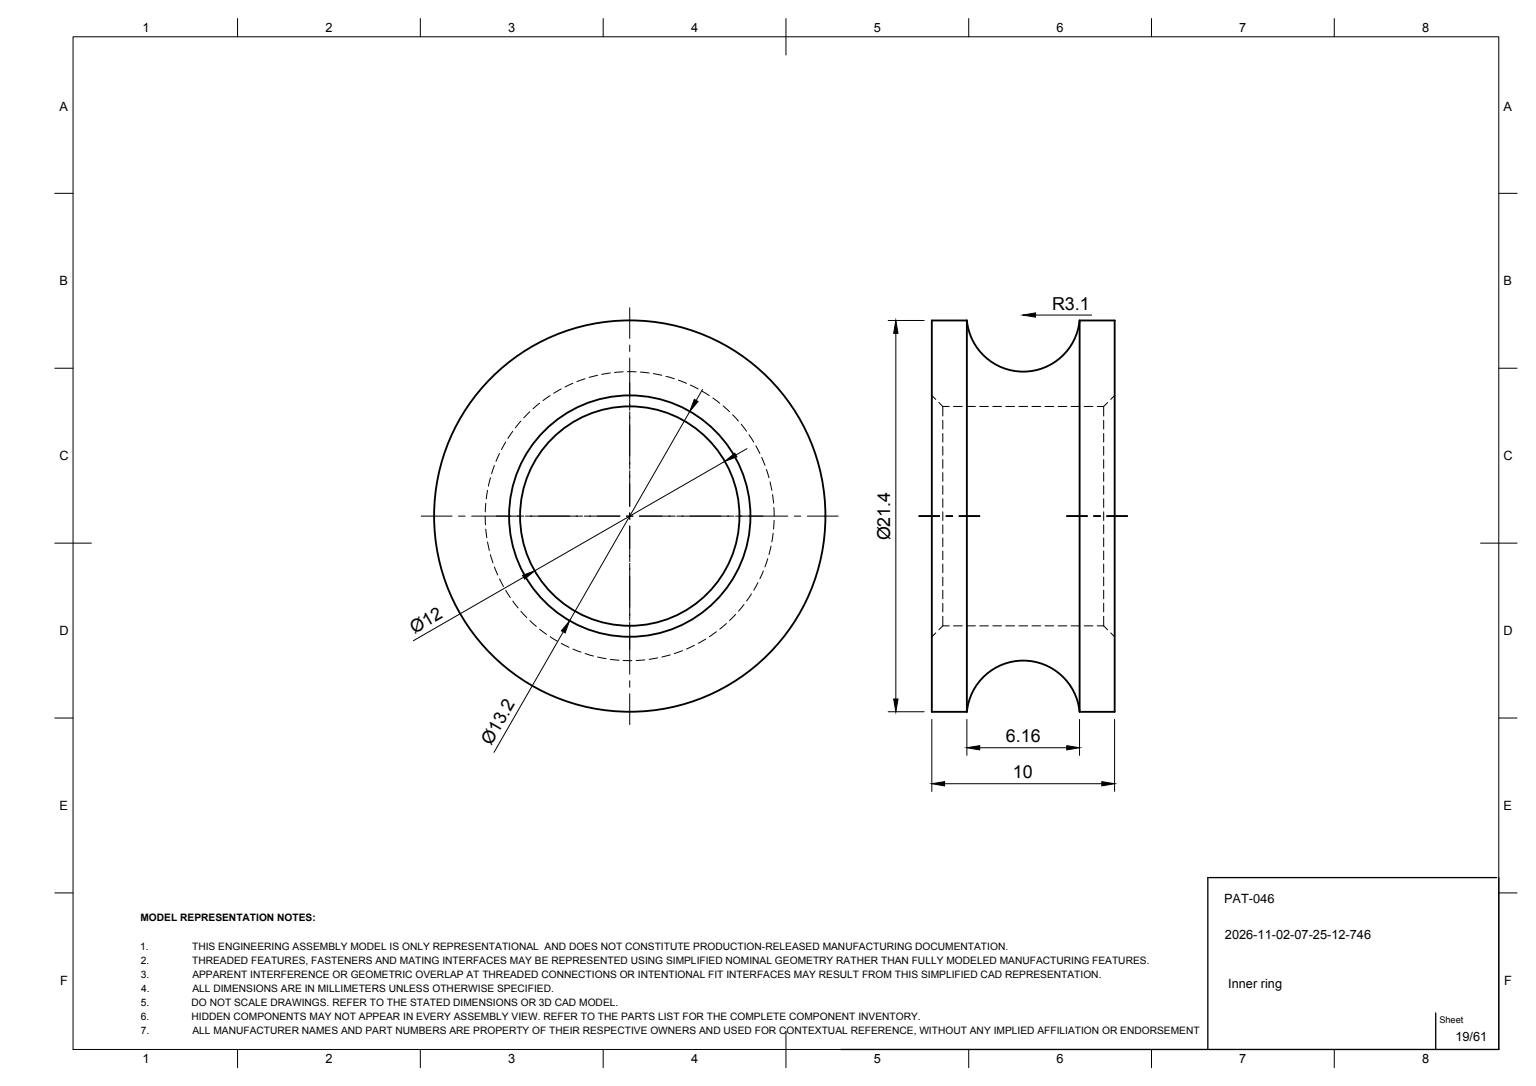
ISO-10303-21;
HEADER;
/* Generated by software containing ST-Developer
 * from STEP Tools, Inc. (www.steptools.com) 
 */

FILE_DESCRIPTION(
/* description */ ('Gear mesh backlash fixture'),
/* implementation_level */ '2;1');

FILE_NAME(
/* name */ 'Inner ring.step',
/* time_stamp */ '2026-10-28T03:26:00-07:00',
/* author */ (''),
/* organization */ (''),
/* preprocessor_version */ 'ST-DEVELOPER v20.2',
/* originating_system */ 'Autodesk Translation Framework v15.17.0.0',
/* authorisation */ '');

FILE_SCHEMA (('AUTOMOTIVE_DESIGN { 1 0 10303 214 3 1 1 }'));
ENDSEC;

DATA;
#10=MECHANICAL_DESIGN_GEOMETRIC_PRESENTATION_REPRESENTATION('',(#1028),#57900);
#759=CONICAL_SURFACE('',#14509,0.63,0.785398163397448);
#760=CONICAL_SURFACE('',#14516,0.63,0.785398163397448);
#780=TOROIDAL_SURFACE('',#14498,1.1,0.309556);
#928=SHAPE_REPRESENTATION_RELATIONSHIP('SRR','None',#58124,#978);
#978=ADVANCED_BREP_SHAPE_REPRESENTATION('',(#1093),#57857);
#1028=STYLED_ITEM('',(#58465),#1093);
#1093=MANIFOLD_SOLID_BREP('Body1',#13588);
#1217=FACE_BOUND('',#2684,.T.);
#1218=FACE_BOUND('',#2687,.T.);
#1413=PLANE('',#14511);
#1414=PLANE('',#14514);
#1840=FACE_OUTER_BOUND('',#2679,.T.);
#1841=FACE_OUTER_BOUND('',#2680,.T.);
#1842=FACE_OUTER_BOUND('',#2681,.T.);
#1843=FACE_OUTER_BOUND('',#2682,.T.);
#1844=FACE_OUTER_BOUND('',#2683,.T.);
#1845=FACE_OUTER_BOUND('',#2685,.T.);
#1846=FACE_OUTER_BOUND('',#2686,.T.);
#1847=FACE_OUTER_BOUND('',#2688,.T.);
#2679=EDGE_LOOP('',(#9547,#9548,#9549,#9550,#9551,#9552));
#2680=EDGE_LOOP('',(#9553,#9554,#9555,#9556,#9557));
#2681=EDGE_LOOP('',(#9558,#9559,#9560,#9561));
#2682=EDGE_LOOP('',(#9562,#9563,#9564,#9565));
#2683=EDGE_LOOP('',(#9566));
#2684=EDGE_LOOP('',(#9567));
#2685=EDGE_LOOP('',(#9568,#9569,#9570,#9571,#9572));
#2686=EDGE_LOOP('',(#9573));
#2687=EDGE_LOOP('',(#9574));
#2688=EDGE_LOOP('',(#9575,#9576,#9577,#9578));
#3597=LINE('',#20054,#4486);
#3598=LINE('',#20060,#4487);
#3599=LINE('',#20064,#4488);
#3600=LINE('',#20070,#4489);
#3601=LINE('',#20075,#4490);
#4486=VECTOR('',#16384,1.070235);
#4487=VECTOR('',#16391,0.6);
#4488=VECTOR('',#16396,0.63);
#4489=VECTOR('',#16405,1.070235);
#4490=VECTOR('',#16412,0.63);
#5330=CIRCLE('',#14499,1.070235);
#5331=CIRCLE('',#14500,1.070235);
#5332=CIRCLE('',#14501,0.309556);
#5333=CIRCLE('',#14502,1.070235);
#5334=CIRCLE('',#14503,1.070235);
#5335=CIRCLE('',#14505,1.070235);
#5336=CIRCLE('',#14507,0.6);
#5337=CIRCLE('',#14508,0.6);
#5338=CIRCLE('',#14510,0.66);
#5339=CIRCLE('',#14513,1.070235);
#5340=CIRCLE('',#14515,0.66);
#5999=VERTEX_POINT('',#20043);
#6000=VERTEX_POINT('',#20044);
#6001=VERTEX_POINT('',#20047);
#6002=VERTEX_POINT('',#20049);
#6003=VERTEX_POINT('',#20053);
#6004=VERTEX_POINT('',#20057);
#6005=VERTEX_POINT('',#20059);
#6006=VERTEX_POINT('',#20063);
#6007=VERTEX_POINT('',#20068);
#6008=VERTEX_POINT('',#20072);
#7360=EDGE_CURVE('',#5999,#6000,#5330,.T.);
#7361=EDGE_CURVE('',#6000,#5999,#5331,.T.);
#7362=EDGE_CURVE('',#6000,#6001,#5332,.T.);
#7363=EDGE_CURVE('',#6002,#6001,#5333,.T.);
#7364=EDGE_CURVE('',#6001,#6002,#5334,.T.);
#7365=EDGE_CURVE('',#6002,#6003,#3597,.T.);
#7366=EDGE_CURVE('',#6003,#6003,#5335,.T.);
#7367=EDGE_CURVE('',#6004,#6004,#5336,.T.);
#7368=EDGE_CURVE('',#6004,#6005,#3598,.T.);
#7369=EDGE_CURVE('',#6005,#6005,#5337,.T.);
#7370=EDGE_CURVE('',#6005,#6006,#3599,.T.);
#7371=EDGE_CURVE('',#6006,#6006,#5338,.T.);
#7372=EDGE_CURVE('',#6007,#6007,#5339,.T.);
#7373=EDGE_CURVE('',#6007,#5999,#3600,.T.);
#7374=EDGE_CURVE('',#6008,#6008,#5340,.T.);
#7375=EDGE_CURVE('',#6008,#6004,#3601,.T.);
#9547=ORIENTED_EDGE('',*,*,#7360,.F.);
#9548=ORIENTED_EDGE('',*,*,#7361,.F.);
#9549=ORIENTED_EDGE('',*,*,#7362,.T.);
#9550=ORIENTED_EDGE('',*,*,#7363,.F.);
#9551=ORIENTED_EDGE('',*,*,#7364,.F.);
#9552=ORIENTED_EDGE('',*,*,#7362,.F.);
#9553=ORIENTED_EDGE('',*,*,#7363,.T.);
#9554=ORIENTED_EDGE('',*,*,#7364,.T.);
#9555=ORIENTED_EDGE('',*,*,#7365,.T.);
#9556=ORIENTED_EDGE('',*,*,#7366,.T.);
#9557=ORIENTED_EDGE('',*,*,#7365,.F.);
#9558=ORIENTED_EDGE('',*,*,#7367,.T.);
#9559=ORIENTED_EDGE('',*,*,#7368,.T.);
#9560=ORIENTED_EDGE('',*,*,#7369,.F.);
#9561=ORIENTED_EDGE('',*,*,#7368,.F.);
#9562=ORIENTED_EDGE('',*,*,#7369,.T.);
#9563=ORIENTED_EDGE('',*,*,#7370,.T.);
#9564=ORIENTED_EDGE('',*,*,#7371,.F.);
#9565=ORIENTED_EDGE('',*,*,#7370,.F.);
#9566=ORIENTED_EDGE('',*,*,#7366,.F.);
#9567=ORIENTED_EDGE('',*,*,#7371,.T.);
#9568=ORIENTED_EDGE('',*,*,#7372,.F.);
#9569=ORIENTED_EDGE('',*,*,#7373,.T.);
#9570=ORIENTED_EDGE('',*,*,#7360,.T.);
#9571=ORIENTED_EDGE('',*,*,#7361,.T.);
#9572=ORIENTED_EDGE('',*,*,#7373,.F.);
#9573=ORIENTED_EDGE('',*,*,#7372,.T.);
#9574=ORIENTED_EDGE('',*,*,#7374,.F.);
#9575=ORIENTED_EDGE('',*,*,#7374,.T.);
#9576=ORIENTED_EDGE('',*,*,#7375,.T.);
#9577=ORIENTED_EDGE('',*,*,#7367,.F.);
#9578=ORIENTED_EDGE('',*,*,#7375,.F.);
#12648=CYLINDRICAL_SURFACE('',#14504,1.070235);
#12649=CYLINDRICAL_SURFACE('',#14506,0.6);
#12650=CYLINDRICAL_SURFACE('',#14512,1.070235);
#12957=ADVANCED_FACE('',(#1840),#780,.F.);
#12958=ADVANCED_FACE('',(#1841),#12648,.T.);
#12959=ADVANCED_FACE('',(#1842),#12649,.F.);
#12960=ADVANCED_FACE('',(#1843),#759,.F.);
#12961=ADVANCED_FACE('',(#1844,#1217),#1413,.T.);
#12962=ADVANCED_FACE('',(#1845),#12650,.T.);
#12963=ADVANCED_FACE('',(#1846,#1218),#1414,.T.);
#12964=ADVANCED_FACE('',(#1847),#760,.F.);
#13588=CLOSED_SHELL('',(#12957,#12958,#12959,#12960,#12961,#12962,#12963,
#12964));
#14497=AXIS2_PLACEMENT_3D('',#20041,#16368,#16369);
#14498=AXIS2_PLACEMENT_3D('',#20042,#16370,#16371);
#14499=AXIS2_PLACEMENT_3D('',#20045,#16372,#16373);
#14500=AXIS2_PLACEMENT_3D('',#20046,#16374,#16375);
#14501=AXIS2_PLACEMENT_3D('',#20048,#16376,#16377);
#14502=AXIS2_PLACEMENT_3D('',#20050,#16378,#16379);
#14503=AXIS2_PLACEMENT_3D('',#20051,#16380,#16381);
#14504=AXIS2_PLACEMENT_3D('',#20052,#16382,#16383);
#14505=AXIS2_PLACEMENT_3D('',#20055,#16385,#16386);
#14506=AXIS2_PLACEMENT_3D('',#20056,#16387,#16388);
#14507=AXIS2_PLACEMENT_3D('',#20058,#16389,#16390);
#14508=AXIS2_PLACEMENT_3D('',#20061,#16392,#16393);
#14509=AXIS2_PLACEMENT_3D('',#20062,#16394,#16395);
#14510=AXIS2_PLACEMENT_3D('',#20065,#16397,#16398);
#14511=AXIS2_PLACEMENT_3D('',#20066,#16399,#16400);
#14512=AXIS2_PLACEMENT_3D('',#20067,#16401,#16402);
#14513=AXIS2_PLACEMENT_3D('',#20069,#16403,#16404);
#14514=AXIS2_PLACEMENT_3D('',#20071,#16406,#16407);
#14515=AXIS2_PLACEMENT_3D('',#20073,#16408,#16409);
#14516=AXIS2_PLACEMENT_3D('',#20074,#16410,#16411);
#16368=DIRECTION('axis',(0.,0.,1.));
#16369=DIRECTION('refdir',(1.,0.,0.));
#16370=DIRECTION('center_axis',(0.,-1.,0.));
#16371=DIRECTION('ref_axis',(0.,0.,-1.));
#16372=DIRECTION('center_axis',(0.,-1.,0.));
#16373=DIRECTION('ref_axis',(1.,0.,0.));
#16374=DIRECTION('center_axis',(0.,-1.,0.));
#16375=DIRECTION('ref_axis',(1.,0.,0.));
#16376=DIRECTION('center_axis',(1.,0.,1.22464679914735E-16));
#16377=DIRECTION('ref_axis',(-1.22464679914735E-16,0.,1.));
#16378=DIRECTION('center_axis',(0.,1.,0.));
#16379=DIRECTION('ref_axis',(1.,0.,0.));
#16380=DIRECTION('center_axis',(0.,1.,0.));
#16381=DIRECTION('ref_axis',(1.,0.,0.));
#16382=DIRECTION('center_axis',(0.,-1.,0.));
#16383=DIRECTION('ref_axis',(1.,0.,0.));
#16384=DIRECTION('',(0.,1.,0.));
#16385=DIRECTION('center_axis',(0.,-1.,0.));
#16386=DIRECTION('ref_axis',(1.,0.,0.));
#16387=DIRECTION('center_axis',(0.,-1.,0.));
#16388=DIRECTION('ref_axis',(1.,0.,0.));
#16389=DIRECTION('center_axis',(0.,-1.,0.));
#16390=DIRECTION('ref_axis',(1.,0.,0.));
#16391=DIRECTION('',(0.,1.,0.));
#16392=DIRECTION('center_axis',(0.,-1.,0.));
#16393=DIRECTION('ref_axis',(1.,0.,0.));
#16394=DIRECTION('center_axis',(0.,1.,0.));
#16395=DIRECTION('ref_axis',(1.,0.,0.));
#16396=DIRECTION('',(-0.707106781186548,0.707106781186547,-8.65956056235493E-17));
#16397=DIRECTION('center_axis',(0.,-1.,0.));
#16398=DIRECTION('ref_axis',(1.,0.,0.));
#16399=DIRECTION('center_axis',(0.,1.,0.));
#16400=DIRECTION('ref_axis',(0.,0.,1.));
#16401=DIRECTION('center_axis',(0.,-1.,0.));
#16402=DIRECTION('ref_axis',(1.,0.,0.));
#16403=DIRECTION('center_axis',(0.,-1.,0.));
#16404=DIRECTION('ref_axis',(1.,0.,0.));
#16405=DIRECTION('',(0.,1.,0.));
#16406=DIRECTION('center_axis',(0.,-1.,0.));
#16407=DIRECTION('ref_axis',(0.,0.,-1.));
#16408=DIRECTION('center_axis',(0.,-1.,0.));
#16409=DIRECTION('ref_axis',(1.,0.,0.));
#16410=DIRECTION('center_axis',(0.,-1.,0.));
#16411=DIRECTION('ref_axis',(1.,0.,0.));
#16412=DIRECTION('',(0.707106781186548,0.707106781186547,8.65956056235493E-17));
#20041=CARTESIAN_POINT('',(0.,0.,0.));
#20042=CARTESIAN_POINT('Origin',(0.,0.,0.));
#20043=CARTESIAN_POINT('',(-1.070235,-0.308121667383195,-1.31065986708547E-16));
#20044=CARTESIAN_POINT('',(-1.31065986708547E-16,-0.308121667383195,1.070235));
#20045=CARTESIAN_POINT('Origin',(0.,-0.308121667383195,0.));
#20046=CARTESIAN_POINT('Origin',(0.,-0.308121667383195,0.));
#20047=CARTESIAN_POINT('',(-1.31065986708547E-16,0.308121667383195,1.070235));
#20048=CARTESIAN_POINT('Origin',(-1.34711147906209E-16,0.,1.1));
#20049=CARTESIAN_POINT('',(-1.070235,0.308121667383195,1.31065986708547E-16));
#20050=CARTESIAN_POINT('Origin',(0.,0.308121667383195,0.));
#20051=CARTESIAN_POINT('Origin',(0.,0.308121667383195,0.));
#20052=CARTESIAN_POINT('Origin',(0.,0.,0.));
#20053=CARTESIAN_POINT('',(-1.070235,0.5,-1.31065986708547E-16));
#20054=CARTESIAN_POINT('',(-1.070235,0.,-1.31065986708547E-16));
#20055=CARTESIAN_POINT('Origin',(0.,0.5,0.));
#20056=CARTESIAN_POINT('Origin',(0.,0.,0.));
#20057=CARTESIAN_POINT('',(-0.6,-0.44,-7.34788079488412E-17));
#20058=CARTESIAN_POINT('Origin',(0.,-0.44,0.));
#20059=CARTESIAN_POINT('',(-0.6,0.44,-7.34788079488412E-17));
#20060=CARTESIAN_POINT('',(-0.6,0.,-7.34788079488412E-17));
#20061=CARTESIAN_POINT('Origin',(0.,0.44,0.));
#20062=CARTESIAN_POINT('Origin',(0.,0.47,0.));
#20063=CARTESIAN_POINT('',(-0.66,0.5,-8.08266887437253E-17));
#20064=CARTESIAN_POINT('',(-0.63,0.47,-7.71527483462832E-17));
#20065=CARTESIAN_POINT('Origin',(0.,0.5,0.));
#20066=CARTESIAN_POINT('Origin',(1.070235,0.5,0.));
#20067=CARTESIAN_POINT('Origin',(0.,0.,0.));
#20068=CARTESIAN_POINT('',(-1.070235,-0.5,-1.31065986708547E-16));
#20069=CARTESIAN_POINT('Origin',(0.,-0.5,0.));
#20070=CARTESIAN_POINT('',(-1.070235,0.,-1.31065986708547E-16));
#20071=CARTESIAN_POINT('Origin',(0.66,-0.5,0.));
#20072=CARTESIAN_POINT('',(-0.66,-0.5,-8.08266887437253E-17));
#20073=CARTESIAN_POINT('Origin',(0.,-0.5,0.));
#20074=CARTESIAN_POINT('Origin',(0.,-0.47,0.));
#20075=CARTESIAN_POINT('',(-0.63,-0.47,-7.71527483462832E-17));
#57798=UNCERTAINTY_MEASURE_WITH_UNIT(LENGTH_MEASURE(0.001),#57901,
'DISTANCE_ACCURACY_VALUE',
'Maximum model space distance between geometric entities at asserted c
onnectivities');
#57841=UNCERTAINTY_MEASURE_WITH_UNIT(LENGTH_MEASURE(0.001),#57901,
'DISTANCE_ACCURACY_VALUE',
'Maximum model space distance between geometric entities at asserted c
onnectivities');
#57857=(
GEOMETRIC_REPRESENTATION_CONTEXT(3)
GLOBAL_UNCERTAINTY_ASSIGNED_CONTEXT((#57798))
GLOBAL_UNIT_ASSIGNED_CONTEXT((#57901,#57903,#57904))
REPRESENTATION_CONTEXT('','3D')
);
#57900=(
GEOMETRIC_REPRESENTATION_CONTEXT(3)
GLOBAL_UNCERTAINTY_ASSIGNED_CONTEXT((#57841))
GLOBAL_UNIT_ASSIGNED_CONTEXT((#57901,#57903,#57904))
REPRESENTATION_CONTEXT('','3D')
);
#57901=(
LENGTH_UNIT()
NAMED_UNIT(*)
SI_UNIT(.CENTI.,.METRE.)
);
#57903=(
NAMED_UNIT(*)
PLANE_ANGLE_UNIT()
SI_UNIT($,.RADIAN.)
);
#57904=(
NAMED_UNIT(*)
SI_UNIT($,.STERADIAN.)
SOLID_ANGLE_UNIT()
);
#57920=SHAPE_DEFINITION_REPRESENTATION(#57978,#58124);
#57978=PRODUCT_DEFINITION_SHAPE('',$,#58183);
#58124=SHAPE_REPRESENTATION('',(#14497),#57857);
#58167=PRODUCT_DEFINITION_CONTEXT('part definition',#58343,'design');
#58183=PRODUCT_DEFINITION('Inner ring','Inner ring',#58241,#58167);
#58241=PRODUCT_DEFINITION_FORMATION('',$,#58360);
#58343=APPLICATION_CONTEXT(
'Core Data for Automotive Mechanical Design Process');
#58344=PRODUCT_CONTEXT('part definition',#58343,'mechanical');
#58360=PRODUCT('Inner ring','Inner ring','Inner ring',(#58344));
#58459=COLOUR_RGB('Grey',0.48,0.52,0.57);
#58460=FILL_AREA_STYLE_COLOUR('',#58459);
#58461=FILL_AREA_STYLE('',(#58460));
#58462=SURFACE_STYLE_FILL_AREA(#58461);
#58463=SURFACE_SIDE_STYLE('',(#58462));
#58464=SURFACE_STYLE_USAGE(.BOTH.,#58463);
#58465=PRESENTATION_STYLE_ASSIGNMENT((#58464));
ENDSEC;
END-ISO-10303-21;
